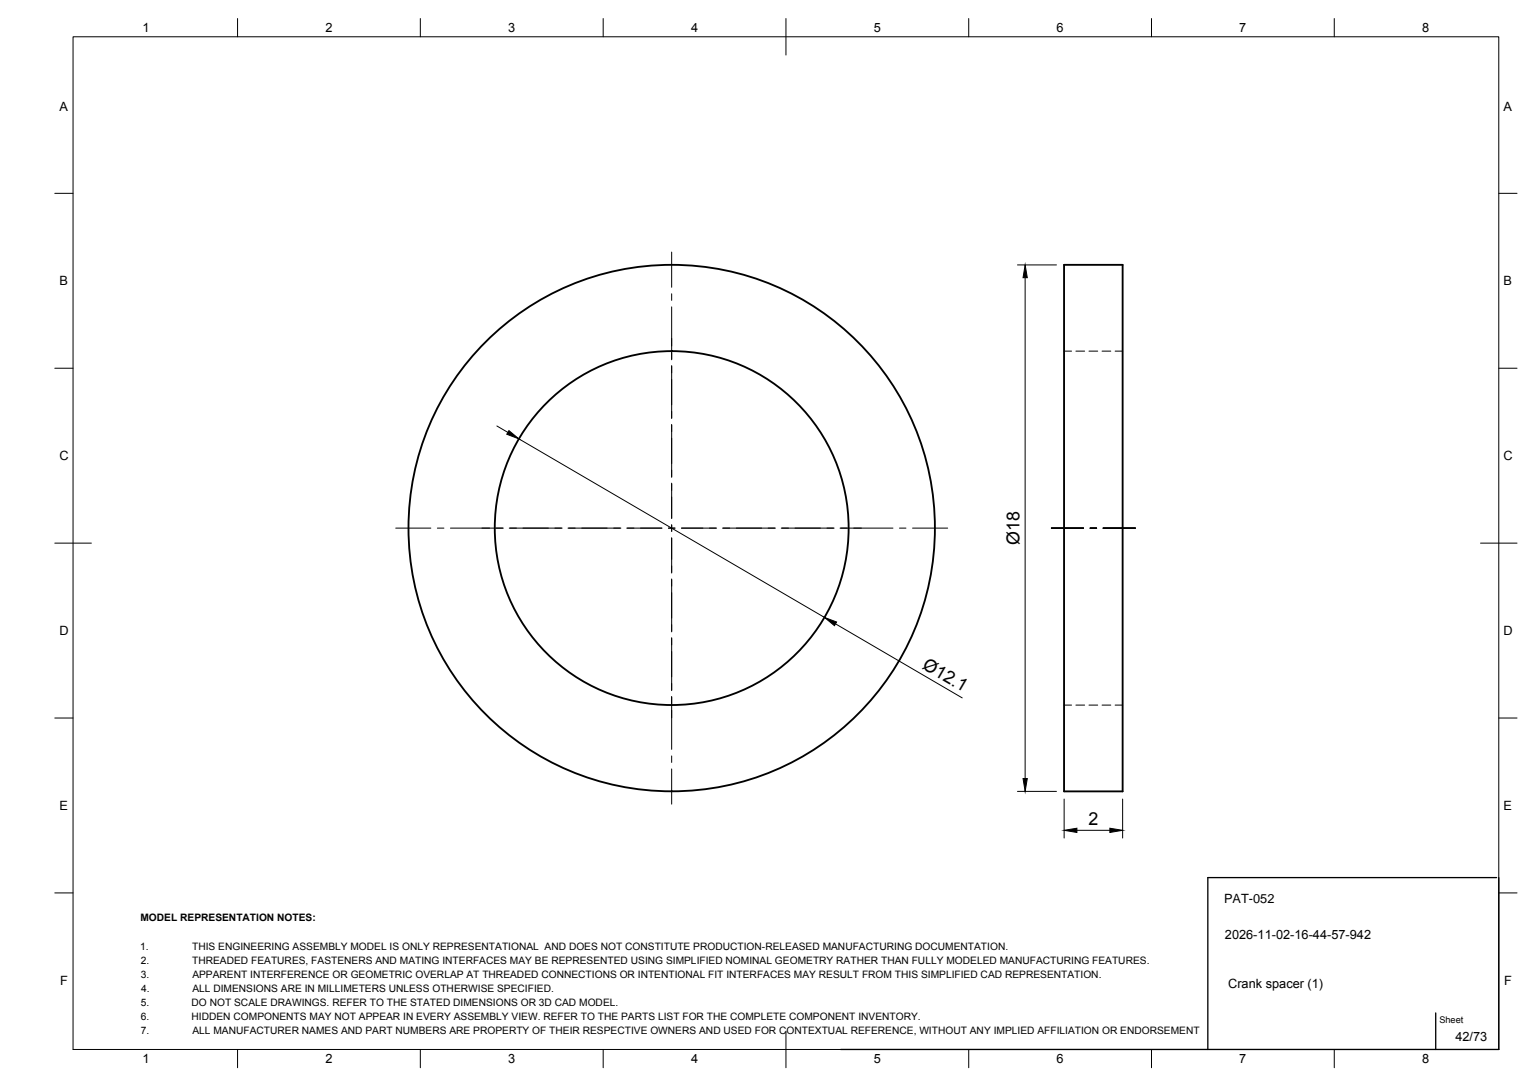
ISO-10303-21;
HEADER;
/* Generated by software containing ST-Developer
 * from STEP Tools, Inc. (www.steptools.com) 
 */

FILE_DESCRIPTION(
/* description */ ('Hand-crank gear train demonstrator'),
/* implementation_level */ '2;1');

FILE_NAME(
/* name */ 'Crank spacer (1).step',
/* time_stamp */ '2026-10-28T03:22:13-07:00',
/* author */ (''),
/* organization */ (''),
/* preprocessor_version */ 'ST-DEVELOPER v20.2',
/* originating_system */ 'Autodesk Translation Framework v15.17.0.0',
/* authorisation */ '');

FILE_SCHEMA (('AUTOMOTIVE_DESIGN { 1 0 10303 214 3 1 1 }'));
ENDSEC;

DATA;
#10=MECHANICAL_DESIGN_GEOMETRIC_PRESENTATION_REPRESENTATION('',(#1238),#62758);
#1095=SHAPE_REPRESENTATION_RELATIONSHIP('SRR','None',#63070,#1159);
#1159=ADVANCED_BREP_SHAPE_REPRESENTATION('',(#1314),#62724);
#1238=STYLED_ITEM('',(#63455),#1314);
#1314=MANIFOLD_SOLID_BREP('Body1',#16421);
#1562=FACE_BOUND('',#3757,.T.);
#1563=FACE_BOUND('',#3759,.T.);
#1917=PLANE('',#18078);
#1918=PLANE('',#18079);
#2598=FACE_OUTER_BOUND('',#3754,.T.);
#2599=FACE_OUTER_BOUND('',#3755,.T.);
#2600=FACE_OUTER_BOUND('',#3756,.T.);
#2601=FACE_OUTER_BOUND('',#3758,.T.);
#3754=EDGE_LOOP('',(#12909,#12910,#12911,#12912));
#3755=EDGE_LOOP('',(#12913,#12914,#12915,#12916));
#3756=EDGE_LOOP('',(#12917));
#3757=EDGE_LOOP('',(#12918));
#3758=EDGE_LOOP('',(#12919));
#3759=EDGE_LOOP('',(#12920));
#4898=LINE('',#26265,#6030);
#4899=LINE('',#26271,#6031);
#6030=VECTOR('',#21275,0.605);
#6031=VECTOR('',#21282,0.9);
#6939=CIRCLE('',#18073,0.605);
#6940=CIRCLE('',#18074,0.605);
#6941=CIRCLE('',#18076,0.9);
#6942=CIRCLE('',#18077,0.9);
#7918=VERTEX_POINT('',#26262);
#7919=VERTEX_POINT('',#26264);
#7920=VERTEX_POINT('',#26268);
#7921=VERTEX_POINT('',#26270);
#9706=EDGE_CURVE('',#7918,#7918,#6939,.T.);
#9707=EDGE_CURVE('',#7918,#7919,#4898,.T.);
#9708=EDGE_CURVE('',#7919,#7919,#6940,.T.);
#9709=EDGE_CURVE('',#7920,#7920,#6941,.T.);
#9710=EDGE_CURVE('',#7920,#7921,#4899,.T.);
#9711=EDGE_CURVE('',#7921,#7921,#6942,.T.);
#12909=ORIENTED_EDGE('',*,*,#9706,.F.);
#12910=ORIENTED_EDGE('',*,*,#9707,.T.);
#12911=ORIENTED_EDGE('',*,*,#9708,.T.);
#12912=ORIENTED_EDGE('',*,*,#9707,.F.);
#12913=ORIENTED_EDGE('',*,*,#9709,.F.);
#12914=ORIENTED_EDGE('',*,*,#9710,.T.);
#12915=ORIENTED_EDGE('',*,*,#9711,.T.);
#12916=ORIENTED_EDGE('',*,*,#9710,.F.);
#12917=ORIENTED_EDGE('',*,*,#9709,.T.);
#12918=ORIENTED_EDGE('',*,*,#9706,.T.);
#12919=ORIENTED_EDGE('',*,*,#9711,.F.);
#12920=ORIENTED_EDGE('',*,*,#9708,.F.);
#15307=CYLINDRICAL_SURFACE('',#18072,0.605);
#15308=CYLINDRICAL_SURFACE('',#18075,0.9);
#15908=ADVANCED_FACE('',(#2598),#15307,.F.);
#15909=ADVANCED_FACE('',(#2599),#15308,.T.);
#15910=ADVANCED_FACE('',(#2600,#1562),#1917,.T.);
#15911=ADVANCED_FACE('',(#2601,#1563),#1918,.F.);
#16421=CLOSED_SHELL('',(#15908,#15909,#15910,#15911));
#18071=AXIS2_PLACEMENT_3D('',#26260,#21269,#21270);
#18072=AXIS2_PLACEMENT_3D('',#26261,#21271,#21272);
#18073=AXIS2_PLACEMENT_3D('',#26263,#21273,#21274);
#18074=AXIS2_PLACEMENT_3D('',#26266,#21276,#21277);
#18075=AXIS2_PLACEMENT_3D('',#26267,#21278,#21279);
#18076=AXIS2_PLACEMENT_3D('',#26269,#21280,#21281);
#18077=AXIS2_PLACEMENT_3D('',#26272,#21283,#21284);
#18078=AXIS2_PLACEMENT_3D('',#26273,#21285,#21286);
#18079=AXIS2_PLACEMENT_3D('',#26274,#21287,#21288);
#21269=DIRECTION('axis',(0.,0.,1.));
#21270=DIRECTION('refdir',(1.,0.,0.));
#21271=DIRECTION('center_axis',(0.,1.,0.));
#21272=DIRECTION('ref_axis',(1.,0.,0.));
#21273=DIRECTION('center_axis',(0.,-1.,0.));
#21274=DIRECTION('ref_axis',(1.,0.,0.));
#21275=DIRECTION('',(0.,-1.,0.));
#21276=DIRECTION('center_axis',(0.,-1.,0.));
#21277=DIRECTION('ref_axis',(1.,0.,0.));
#21278=DIRECTION('center_axis',(0.,1.,0.));
#21279=DIRECTION('ref_axis',(1.,0.,0.));
#21280=DIRECTION('center_axis',(0.,1.,0.));
#21281=DIRECTION('ref_axis',(1.,0.,0.));
#21282=DIRECTION('',(0.,-1.,0.));
#21283=DIRECTION('center_axis',(0.,1.,0.));
#21284=DIRECTION('ref_axis',(1.,0.,0.));
#21285=DIRECTION('center_axis',(0.,1.,0.));
#21286=DIRECTION('ref_axis',(1.,0.,0.));
#21287=DIRECTION('center_axis',(0.,1.,0.));
#21288=DIRECTION('ref_axis',(1.,0.,0.));
#26260=CARTESIAN_POINT('',(0.,0.,0.));
#26261=CARTESIAN_POINT('Origin',(0.,5.8,9.));
#26262=CARTESIAN_POINT('',(-0.605,6.,9.));
#26263=CARTESIAN_POINT('Origin',(0.,6.,9.));
#26264=CARTESIAN_POINT('',(-0.605,5.8,9.));
#26265=CARTESIAN_POINT('',(-0.605,5.8,9.));
#26266=CARTESIAN_POINT('Origin',(0.,5.8,9.));
#26267=CARTESIAN_POINT('Origin',(0.,5.8,9.));
#26268=CARTESIAN_POINT('',(-0.9,6.,9.));
#26269=CARTESIAN_POINT('Origin',(0.,6.,9.));
#26270=CARTESIAN_POINT('',(-0.9,5.8,9.));
#26271=CARTESIAN_POINT('',(-0.9,5.8,9.));
#26272=CARTESIAN_POINT('Origin',(0.,5.8,9.));
#26273=CARTESIAN_POINT('Origin',(0.,6.,9.));
#26274=CARTESIAN_POINT('Origin',(0.,5.8,9.));
#62650=UNCERTAINTY_MEASURE_WITH_UNIT(LENGTH_MEASURE(0.001),#62759,
'DISTANCE_ACCURACY_VALUE',
'Maximum model space distance between geometric entities at asserted c
onnectivities');
#62684=UNCERTAINTY_MEASURE_WITH_UNIT(LENGTH_MEASURE(0.001),#62759,
'DISTANCE_ACCURACY_VALUE',
'Maximum model space distance between geometric entities at asserted c
onnectivities');
#62724=(
GEOMETRIC_REPRESENTATION_CONTEXT(3)
GLOBAL_UNCERTAINTY_ASSIGNED_CONTEXT((#62650))
GLOBAL_UNIT_ASSIGNED_CONTEXT((#62759,#62761,#62762))
REPRESENTATION_CONTEXT('','3D')
);
#62758=(
GEOMETRIC_REPRESENTATION_CONTEXT(3)
GLOBAL_UNCERTAINTY_ASSIGNED_CONTEXT((#62684))
GLOBAL_UNIT_ASSIGNED_CONTEXT((#62759,#62761,#62762))
REPRESENTATION_CONTEXT('','3D')
);
#62759=(
LENGTH_UNIT()
NAMED_UNIT(*)
SI_UNIT(.CENTI.,.METRE.)
);
#62761=(
NAMED_UNIT(*)
PLANE_ANGLE_UNIT()
SI_UNIT($,.RADIAN.)
);
#62762=(
NAMED_UNIT(*)
SI_UNIT($,.STERADIAN.)
SOLID_ANGLE_UNIT()
);
#62802=SHAPE_DEFINITION_REPRESENTATION(#62885,#63070);
#62885=PRODUCT_DEFINITION_SHAPE('',$,#63144);
#63070=SHAPE_REPRESENTATION('',(#18071),#62724);
#63104=PRODUCT_DEFINITION_CONTEXT('part definition',#63325,'design');
#63144=PRODUCT_DEFINITION('Crank spacer (1)','Crank spacer (1)',#63217,#63104);
#63217=PRODUCT_DEFINITION_FORMATION('',$,#63366);
#63325=APPLICATION_CONTEXT(
'Core Data for Automotive Mechanical Design Process');
#63326=PRODUCT_CONTEXT('part definition',#63325,'mechanical');
#63366=PRODUCT('Crank spacer (1)','Crank spacer (1)','Crank spacer (1)',(#63326));
#63449=COLOUR_RGB('Sky Blue',0.24,0.69,0.87);
#63450=FILL_AREA_STYLE_COLOUR('',#63449);
#63451=FILL_AREA_STYLE('',(#63450));
#63452=SURFACE_STYLE_FILL_AREA(#63451);
#63453=SURFACE_SIDE_STYLE('',(#63452));
#63454=SURFACE_STYLE_USAGE(.BOTH.,#63453);
#63455=PRESENTATION_STYLE_ASSIGNMENT((#63454));
ENDSEC;
END-ISO-10303-21;
